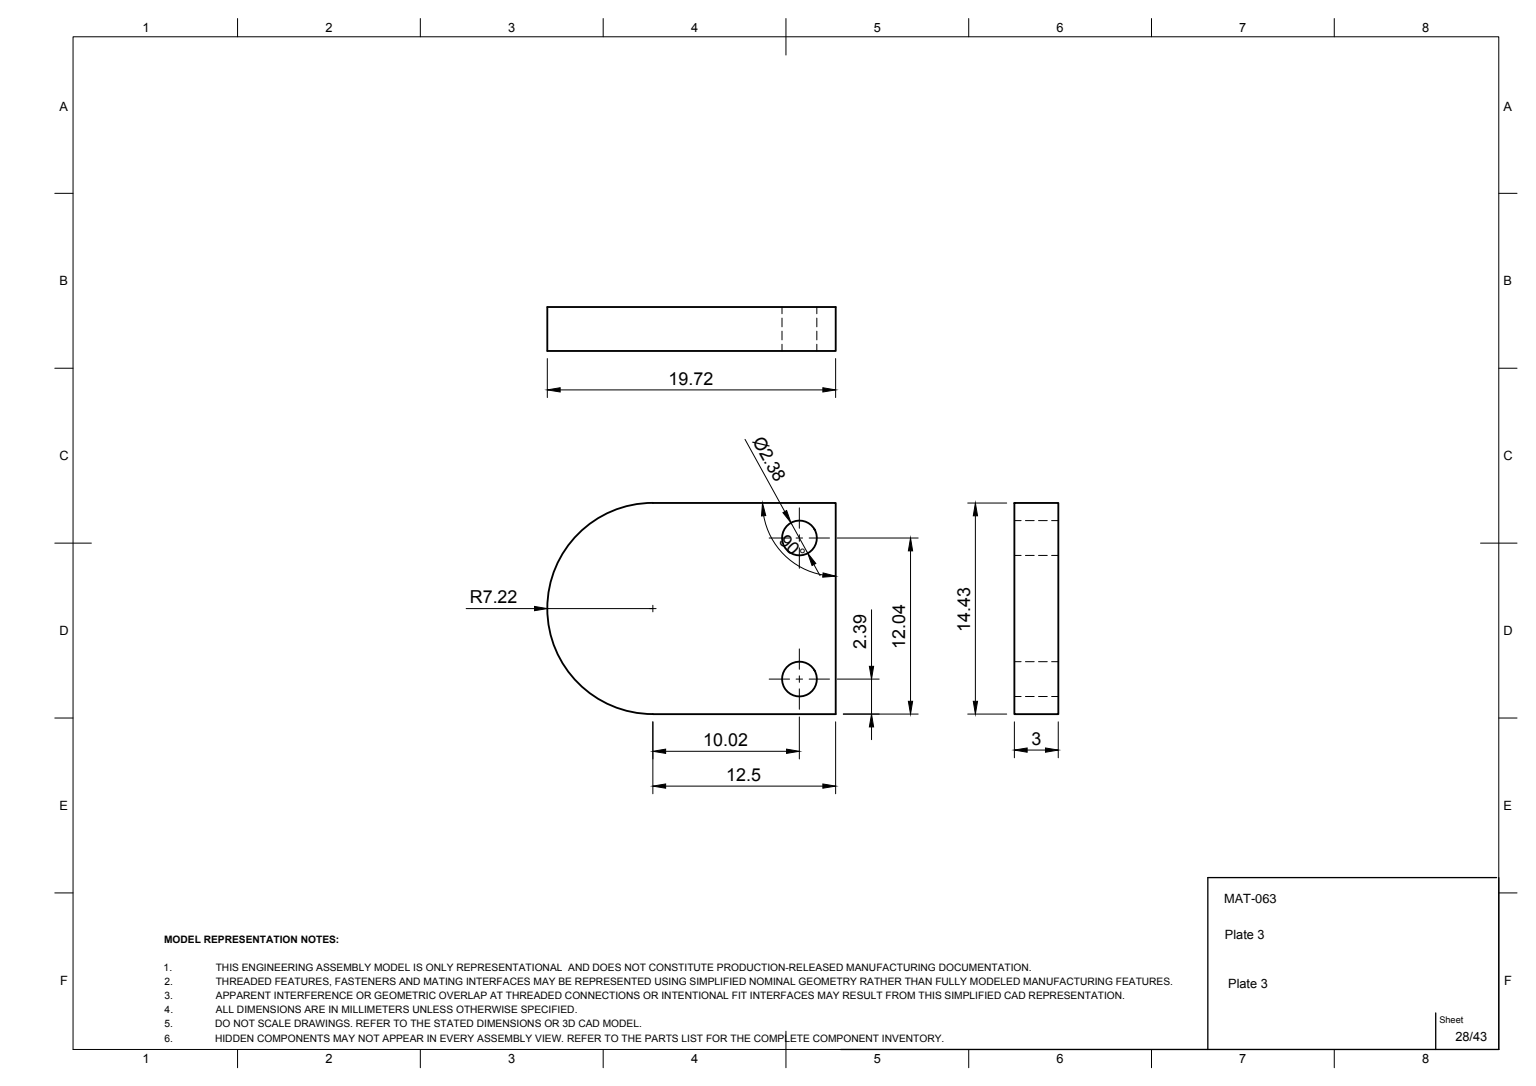
ISO-10303-21;
HEADER;
/* Generated by software containing ST-Developer
 * from STEP Tools, Inc. (www.steptools.com) 
 */

FILE_DESCRIPTION(
/* description */ (''),
/* implementation_level */ '2;1');

FILE_NAME(
/* name */ 'Plate 3.step',
/* time_stamp */ '2026-10-24T09:43:01-07:00',
/* author */ (''),
/* organization */ (''),
/* preprocessor_version */ 'ST-DEVELOPER v20.2',
/* originating_system */ 'Autodesk Translation Framework v15.15.0.0',
/* authorisation */ '');

FILE_SCHEMA (('AUTOMOTIVE_DESIGN { 1 0 10303 214 3 1 1 }'));
ENDSEC;

DATA;
#10=MECHANICAL_DESIGN_GEOMETRIC_PRESENTATION_REPRESENTATION('',(#293),#11112);
#227=SHAPE_REPRESENTATION_RELATIONSHIP('SRR','None',#11252,#260);
#260=ADVANCED_BREP_SHAPE_REPRESENTATION('',(#326),#11097);
#293=STYLED_ITEM('',(#11426),#326);
#326=MANIFOLD_SOLID_BREP('Plate 3',#6030);
#459=FACE_BOUND('',#1443,.T.);
#460=FACE_BOUND('',#1444,.T.);
#461=FACE_BOUND('',#1451,.T.);
#462=FACE_BOUND('',#1452,.T.);
#621=PLANE('',#7071);
#622=PLANE('',#7076);
#623=PLANE('',#7079);
#624=PLANE('',#7080);
#625=PLANE('',#7081);
#957=FACE_OUTER_BOUND('',#1441,.T.);
#958=FACE_OUTER_BOUND('',#1442,.T.);
#959=FACE_OUTER_BOUND('',#1445,.T.);
#960=FACE_OUTER_BOUND('',#1446,.T.);
#961=FACE_OUTER_BOUND('',#1447,.T.);
#962=FACE_OUTER_BOUND('',#1448,.T.);
#963=FACE_OUTER_BOUND('',#1449,.T.);
#964=FACE_OUTER_BOUND('',#1450,.T.);
#1441=EDGE_LOOP('',(#5173,#5174,#5175,#5176));
#1442=EDGE_LOOP('',(#5177,#5178,#5179,#5180));
#1443=EDGE_LOOP('',(#5181));
#1444=EDGE_LOOP('',(#5182));
#1445=EDGE_LOOP('',(#5183,#5184,#5185,#5186));
#1446=EDGE_LOOP('',(#5187,#5188,#5189,#5190));
#1447=EDGE_LOOP('',(#5191,#5192,#5193,#5194));
#1448=EDGE_LOOP('',(#5195,#5196,#5197,#5198));
#1449=EDGE_LOOP('',(#5199,#5200,#5201,#5202));
#1450=EDGE_LOOP('',(#5203,#5204,#5205,#5206));
#1451=EDGE_LOOP('',(#5207));
#1452=EDGE_LOOP('',(#5208));
#1822=LINE('',#10642,#2181);
#1823=LINE('',#10647,#2182);
#1824=LINE('',#10649,#2183);
#1825=LINE('',#10652,#2184);
#1826=LINE('',#10657,#2185);
#1827=LINE('',#10661,#2186);
#1828=LINE('',#10663,#2187);
#1829=LINE('',#10664,#2188);
#1830=LINE('',#10667,#2189);
#1831=LINE('',#10671,#2190);
#1832=LINE('',#10672,#2191);
#1833=LINE('',#10674,#2192);
#2181=VECTOR('',#8850,0.00118970000000007);
#2182=VECTOR('',#8855,0.01);
#2183=VECTOR('',#8856,0.01);
#2184=VECTOR('',#8859,0.01);
#2185=VECTOR('',#8864,0.00118970100000004);
#2186=VECTOR('',#8869,0.01);
#2187=VECTOR('',#8870,0.01);
#2188=VECTOR('',#8871,0.01);
#2189=VECTOR('',#8874,0.01);
#2190=VECTOR('',#8879,0.01);
#2191=VECTOR('',#8880,0.01);
#2192=VECTOR('',#8883,0.01);
#2622=CIRCLE('',#7069,0.00118970000000007);
#2623=CIRCLE('',#7070,0.00118970000000007);
#2624=CIRCLE('',#7072,0.007216878);
#2625=CIRCLE('',#7073,0.00118970100000004);
#2626=CIRCLE('',#7075,0.00118970100000004);
#2627=CIRCLE('',#7078,0.007216878);
#3070=VERTEX_POINT('',#10639);
#3071=VERTEX_POINT('',#10641);
#3072=VERTEX_POINT('',#10645);
#3073=VERTEX_POINT('',#10646);
#3074=VERTEX_POINT('',#10648);
#3075=VERTEX_POINT('',#10650);
#3076=VERTEX_POINT('',#10653);
#3077=VERTEX_POINT('',#10656);
#3078=VERTEX_POINT('',#10660);
#3079=VERTEX_POINT('',#10662);
#3080=VERTEX_POINT('',#10666);
#3081=VERTEX_POINT('',#10670);
#3790=EDGE_CURVE('',#3070,#3070,#2622,.T.);
#3791=EDGE_CURVE('',#3070,#3071,#1822,.T.);
#3792=EDGE_CURVE('',#3071,#3071,#2623,.F.);
#3793=EDGE_CURVE('',#3072,#3073,#1823,.T.);
#3794=EDGE_CURVE('',#3073,#3074,#1824,.T.);
#3795=EDGE_CURVE('',#3074,#3075,#2624,.F.);
#3796=EDGE_CURVE('',#3075,#3072,#1825,.T.);
#3797=EDGE_CURVE('',#3076,#3076,#2625,.T.);
#3798=EDGE_CURVE('',#3076,#3077,#1826,.T.);
#3799=EDGE_CURVE('',#3077,#3077,#2626,.F.);
#3800=EDGE_CURVE('',#3078,#3075,#1827,.T.);
#3801=EDGE_CURVE('',#3079,#3078,#1828,.T.);
#3802=EDGE_CURVE('',#3072,#3079,#1829,.T.);
#3803=EDGE_CURVE('',#3074,#3080,#1830,.F.);
#3804=EDGE_CURVE('',#3080,#3078,#2627,.F.);
#3805=EDGE_CURVE('',#3081,#3073,#1831,.T.);
#3806=EDGE_CURVE('',#3080,#3081,#1832,.T.);
#3807=EDGE_CURVE('',#3081,#3079,#1833,.T.);
#5173=ORIENTED_EDGE('',*,*,#3790,.F.);
#5174=ORIENTED_EDGE('',*,*,#3791,.T.);
#5175=ORIENTED_EDGE('',*,*,#3792,.F.);
#5176=ORIENTED_EDGE('',*,*,#3791,.F.);
#5177=ORIENTED_EDGE('',*,*,#3793,.T.);
#5178=ORIENTED_EDGE('',*,*,#3794,.T.);
#5179=ORIENTED_EDGE('',*,*,#3795,.T.);
#5180=ORIENTED_EDGE('',*,*,#3796,.T.);
#5181=ORIENTED_EDGE('',*,*,#3797,.T.);
#5182=ORIENTED_EDGE('',*,*,#3790,.T.);
#5183=ORIENTED_EDGE('',*,*,#3797,.F.);
#5184=ORIENTED_EDGE('',*,*,#3798,.T.);
#5185=ORIENTED_EDGE('',*,*,#3799,.F.);
#5186=ORIENTED_EDGE('',*,*,#3798,.F.);
#5187=ORIENTED_EDGE('',*,*,#3800,.F.);
#5188=ORIENTED_EDGE('',*,*,#3801,.F.);
#5189=ORIENTED_EDGE('',*,*,#3802,.F.);
#5190=ORIENTED_EDGE('',*,*,#3796,.F.);
#5191=ORIENTED_EDGE('',*,*,#3803,.T.);
#5192=ORIENTED_EDGE('',*,*,#3804,.T.);
#5193=ORIENTED_EDGE('',*,*,#3800,.T.);
#5194=ORIENTED_EDGE('',*,*,#3795,.F.);
#5195=ORIENTED_EDGE('',*,*,#3805,.F.);
#5196=ORIENTED_EDGE('',*,*,#3806,.F.);
#5197=ORIENTED_EDGE('',*,*,#3803,.F.);
#5198=ORIENTED_EDGE('',*,*,#3794,.F.);
#5199=ORIENTED_EDGE('',*,*,#3802,.T.);
#5200=ORIENTED_EDGE('',*,*,#3807,.F.);
#5201=ORIENTED_EDGE('',*,*,#3805,.T.);
#5202=ORIENTED_EDGE('',*,*,#3793,.F.);
#5203=ORIENTED_EDGE('',*,*,#3806,.T.);
#5204=ORIENTED_EDGE('',*,*,#3807,.T.);
#5205=ORIENTED_EDGE('',*,*,#3801,.T.);
#5206=ORIENTED_EDGE('',*,*,#3804,.F.);
#5207=ORIENTED_EDGE('',*,*,#3799,.T.);
#5208=ORIENTED_EDGE('',*,*,#3792,.T.);
#5610=CYLINDRICAL_SURFACE('',#7068,0.00118970000000007);
#5611=CYLINDRICAL_SURFACE('',#7074,0.00118970100000004);
#5612=CYLINDRICAL_SURFACE('',#7077,0.007216878);
#5930=ADVANCED_FACE('',(#957),#5610,.F.);
#5931=ADVANCED_FACE('',(#958,#459,#460),#621,.T.);
#5932=ADVANCED_FACE('',(#959),#5611,.F.);
#5933=ADVANCED_FACE('',(#960),#622,.F.);
#5934=ADVANCED_FACE('',(#961),#5612,.T.);
#5935=ADVANCED_FACE('',(#962),#623,.F.);
#5936=ADVANCED_FACE('',(#963),#624,.F.);
#5937=ADVANCED_FACE('',(#964,#461,#462),#625,.F.);
#6030=CLOSED_SHELL('',(#5930,#5931,#5932,#5933,#5934,#5935,#5936,#5937));
#7067=AXIS2_PLACEMENT_3D('',#10637,#8844,#8845);
#7068=AXIS2_PLACEMENT_3D('',#10638,#8846,#8847);
#7069=AXIS2_PLACEMENT_3D('',#10640,#8848,#8849);
#7070=AXIS2_PLACEMENT_3D('',#10643,#8851,#8852);
#7071=AXIS2_PLACEMENT_3D('',#10644,#8853,#8854);
#7072=AXIS2_PLACEMENT_3D('',#10651,#8857,#8858);
#7073=AXIS2_PLACEMENT_3D('',#10654,#8860,#8861);
#7074=AXIS2_PLACEMENT_3D('',#10655,#8862,#8863);
#7075=AXIS2_PLACEMENT_3D('',#10658,#8865,#8866);
#7076=AXIS2_PLACEMENT_3D('',#10659,#8867,#8868);
#7077=AXIS2_PLACEMENT_3D('',#10665,#8872,#8873);
#7078=AXIS2_PLACEMENT_3D('',#10668,#8875,#8876);
#7079=AXIS2_PLACEMENT_3D('',#10669,#8877,#8878);
#7080=AXIS2_PLACEMENT_3D('',#10673,#8881,#8882);
#7081=AXIS2_PLACEMENT_3D('',#10675,#8884,#8885);
#8844=DIRECTION('axis',(0.,0.,1.));
#8845=DIRECTION('refdir',(1.,0.,0.));
#8846=DIRECTION('center_axis',(1.,0.,0.));
#8847=DIRECTION('ref_axis',(0.,0.,-1.));
#8848=DIRECTION('center_axis',(1.,0.,0.));
#8849=DIRECTION('ref_axis',(0.,0.,-1.));
#8850=DIRECTION('',(1.,0.,0.));
#8851=DIRECTION('center_axis',(1.,0.,0.));
#8852=DIRECTION('ref_axis',(0.,0.,-1.));
#8853=DIRECTION('center_axis',(-1.,3.89528313543134E-16,9.13571080051068E-16));
#8854=DIRECTION('ref_axis',(9.13571080051068E-16,0.,1.));
#8855=DIRECTION('',(0.,0.499999981040771,-0.866025414730555));
#8856=DIRECTION('',(0.,-0.866025392838329,-0.500000018959218));
#8857=DIRECTION('center_axis',(1.,0.,0.));
#8858=DIRECTION('ref_axis',(0.,0.,-1.));
#8859=DIRECTION('',(1.1368683753664E-14,0.866025412838334,0.499999984318194));
#8860=DIRECTION('center_axis',(1.,0.,0.));
#8861=DIRECTION('ref_axis',(0.,0.,-1.));
#8862=DIRECTION('center_axis',(1.,0.,0.));
#8863=DIRECTION('ref_axis',(0.,0.,-1.));
#8864=DIRECTION('',(1.,0.,0.));
#8865=DIRECTION('center_axis',(1.,0.,0.));
#8866=DIRECTION('ref_axis',(0.,0.,-1.));
#8867=DIRECTION('center_axis',(1.0385048021943E-14,0.499999984318195,-0.866025412838333));
#8868=DIRECTION('ref_axis',(-5.27128262282187E-31,0.866025412838333,0.499999984318195));
#8869=DIRECTION('',(-1.,0.,0.));
#8870=DIRECTION('',(0.,-0.866025412838314,-0.499999984318228));
#8871=DIRECTION('',(1.,0.,0.));
#8872=DIRECTION('center_axis',(1.,0.,0.));
#8873=DIRECTION('ref_axis',(0.,0.,-1.));
#8874=DIRECTION('',(-1.,0.,0.));
#8875=DIRECTION('center_axis',(1.,0.,0.));
#8876=DIRECTION('ref_axis',(0.,0.,-1.));
#8877=DIRECTION('center_axis',(-3.97614054718644E-15,-0.500000018959218,
0.866025392838329));
#8878=DIRECTION('ref_axis',(3.1172350974474E-31,-0.866025392838329,-0.500000018959218));
#8879=DIRECTION('',(-1.,0.,0.));
#8880=DIRECTION('',(0.,0.866025392838324,0.500000018959226));
#8881=DIRECTION('center_axis',(6.40929678096138E-15,-0.866025414730554,
-0.499999981040772));
#8882=DIRECTION('ref_axis',(-1.92466517757951E-31,0.499999981040772,-0.866025414730554));
#8883=DIRECTION('',(0.,-0.499999981040781,0.866025414730549));
#8884=DIRECTION('center_axis',(-1.,-7.461387415107E-16,2.73067399557772E-16));
#8885=DIRECTION('ref_axis',(7.461387415107E-16,-1.,9.62450997316976E-49));
#10637=CARTESIAN_POINT('',(0.,0.,0.));
#10638=CARTESIAN_POINT('Origin',(-0.493,-0.542782557,0.975695518));
#10639=CARTESIAN_POINT('',(-0.493,-0.542782557,0.976885218));
#10640=CARTESIAN_POINT('Origin',(-0.493,-0.542782557,0.975695518));
#10641=CARTESIAN_POINT('',(-0.49,-0.542782557,0.976885218));
#10642=CARTESIAN_POINT('',(-0.493,-0.542782557,0.976885218));
#10643=CARTESIAN_POINT('Origin',(-0.49,-0.542782557,0.975695518));
#10644=CARTESIAN_POINT('Origin',(-0.493,-0.545454380845136,0.969136388159038));
#10645=CARTESIAN_POINT('',(-0.493,-0.541830423000466,0.979010345999528));
#10646=CARTESIAN_POINT('',(-0.493,-0.534613544999688,0.966510345999423));
#10647=CARTESIAN_POINT('',(-0.493,-0.541830422948787,0.979010345911298));
#10648=CARTESIAN_POINT('',(-0.492999999983539,-0.545438861934028,0.9602603461963));
#10649=CARTESIAN_POINT('',(-0.493,-0.534613545009254,0.966510345994658));
#10650=CARTESIAN_POINT('',(-0.493,-0.552655740808602,0.972760345664227));
#10651=CARTESIAN_POINT('Origin',(-0.493,-0.549047301,0.966510346));
#10652=CARTESIAN_POINT('',(-0.493,-0.552655741001846,0.972760345998934));
#10653=CARTESIAN_POINT('',(-0.493,-0.537960337,0.968532889));
#10654=CARTESIAN_POINT('Origin',(-0.493,-0.537960337,0.967343188));
#10655=CARTESIAN_POINT('Origin',(-0.493,-0.537960337,0.967343188));
#10656=CARTESIAN_POINT('',(-0.49,-0.537960337,0.968532889));
#10657=CARTESIAN_POINT('',(-0.493,-0.537960337,0.968532889));
#10658=CARTESIAN_POINT('Origin',(-0.49,-0.537960337,0.967343188));
#10659=CARTESIAN_POINT('Origin',(-0.4915,-0.547243082,0.975885346));
#10660=CARTESIAN_POINT('',(-0.49,-0.552655740613422,0.972760345925411));
#10661=CARTESIAN_POINT('',(-0.49,-0.552655741,0.972760346));
#10662=CARTESIAN_POINT('',(-0.49,-0.541830423,0.979010346));
#10663=CARTESIAN_POINT('',(-0.49,-0.541830423,0.979010346));
#10664=CARTESIAN_POINT('',(-0.493,-0.541830423,0.979010346));
#10665=CARTESIAN_POINT('Origin',(-0.493,-0.549047301,0.966510346));
#10666=CARTESIAN_POINT('',(-0.49,-0.54543886200176,0.960260346156978));
#10667=CARTESIAN_POINT('',(-0.49000000025,-0.545438862001176,0.960260346315308));
#10668=CARTESIAN_POINT('Origin',(-0.49,-0.549047301,0.966510346));
#10669=CARTESIAN_POINT('Origin',(-0.4915,-0.5400262035,0.963385346000001));
#10670=CARTESIAN_POINT('',(-0.49,-0.534613545,0.966510346));
#10671=CARTESIAN_POINT('',(-0.49,-0.534613545,0.966510346000001));
#10672=CARTESIAN_POINT('',(-0.49,-0.545438861933347,0.960260346038483));
#10673=CARTESIAN_POINT('Origin',(-0.4915,-0.538221983999999,0.972760345999999));
#10674=CARTESIAN_POINT('',(-0.49,-0.534613544999999,0.966510346));
#10675=CARTESIAN_POINT('Origin',(-0.49,-0.545454380845136,0.969136388159038));
#11058=UNCERTAINTY_MEASURE_WITH_UNIT(LENGTH_MEASURE(1.E-5),#11113,
'DISTANCE_ACCURACY_VALUE',
'Maximum model space distance between geometric entities at asserted c
onnectivities');
#11073=UNCERTAINTY_MEASURE_WITH_UNIT(LENGTH_MEASURE(1.E-5),#11113,
'DISTANCE_ACCURACY_VALUE',
'Maximum model space distance between geometric entities at asserted c
onnectivities');
#11097=(
GEOMETRIC_REPRESENTATION_CONTEXT(3)
GLOBAL_UNCERTAINTY_ASSIGNED_CONTEXT((#11058))
GLOBAL_UNIT_ASSIGNED_CONTEXT((#11113,#11114,#11115))
REPRESENTATION_CONTEXT('','3D')
);
#11112=(
GEOMETRIC_REPRESENTATION_CONTEXT(3)
GLOBAL_UNCERTAINTY_ASSIGNED_CONTEXT((#11073))
GLOBAL_UNIT_ASSIGNED_CONTEXT((#11113,#11114,#11115))
REPRESENTATION_CONTEXT('','3D')
);
#11113=(
LENGTH_UNIT()
NAMED_UNIT(*)
SI_UNIT($,.METRE.)
);
#11114=(
NAMED_UNIT(*)
PLANE_ANGLE_UNIT()
SI_UNIT($,.RADIAN.)
);
#11115=(
NAMED_UNIT(*)
SI_UNIT($,.STERADIAN.)
SOLID_ANGLE_UNIT()
);
#11139=SHAPE_DEFINITION_REPRESENTATION(#11184,#11252);
#11184=PRODUCT_DEFINITION_SHAPE('',$,#11291);
#11252=SHAPE_REPRESENTATION('',(#7067),#11097);
#11267=PRODUCT_DEFINITION_CONTEXT('part definition',#11383,'design');
#11291=PRODUCT_DEFINITION('Plate 3','Plate 3',#11329,#11267);
#11329=PRODUCT_DEFINITION_FORMATION('',$,#11408);
#11383=APPLICATION_CONTEXT(
'Core Data for Automotive Mechanical Design Process');
#11384=PRODUCT_CONTEXT('part definition',#11383,'mechanical');
#11408=PRODUCT('Plate 3','Plate 3','all_plates__ DE      811',(#11384));
#11426=PRESENTATION_STYLE_ASSIGNMENT((#11430));
#11430=SURFACE_STYLE_USAGE(.BOTH.,#11434);
#11434=SURFACE_SIDE_STYLE('',(#11438));
#11438=SURFACE_STYLE_FILL_AREA(#11442);
#11442=FILL_AREA_STYLE('Opaque(202,209,238)',(#11446));
#11446=FILL_AREA_STYLE_COLOUR('Opaque(202,209,238)',#11450);
#11450=COLOUR_RGB('Opaque(202,209,238)',0.792156862745098,0.819607843137255,
0.933333333333333);
ENDSEC;
END-ISO-10303-21;
